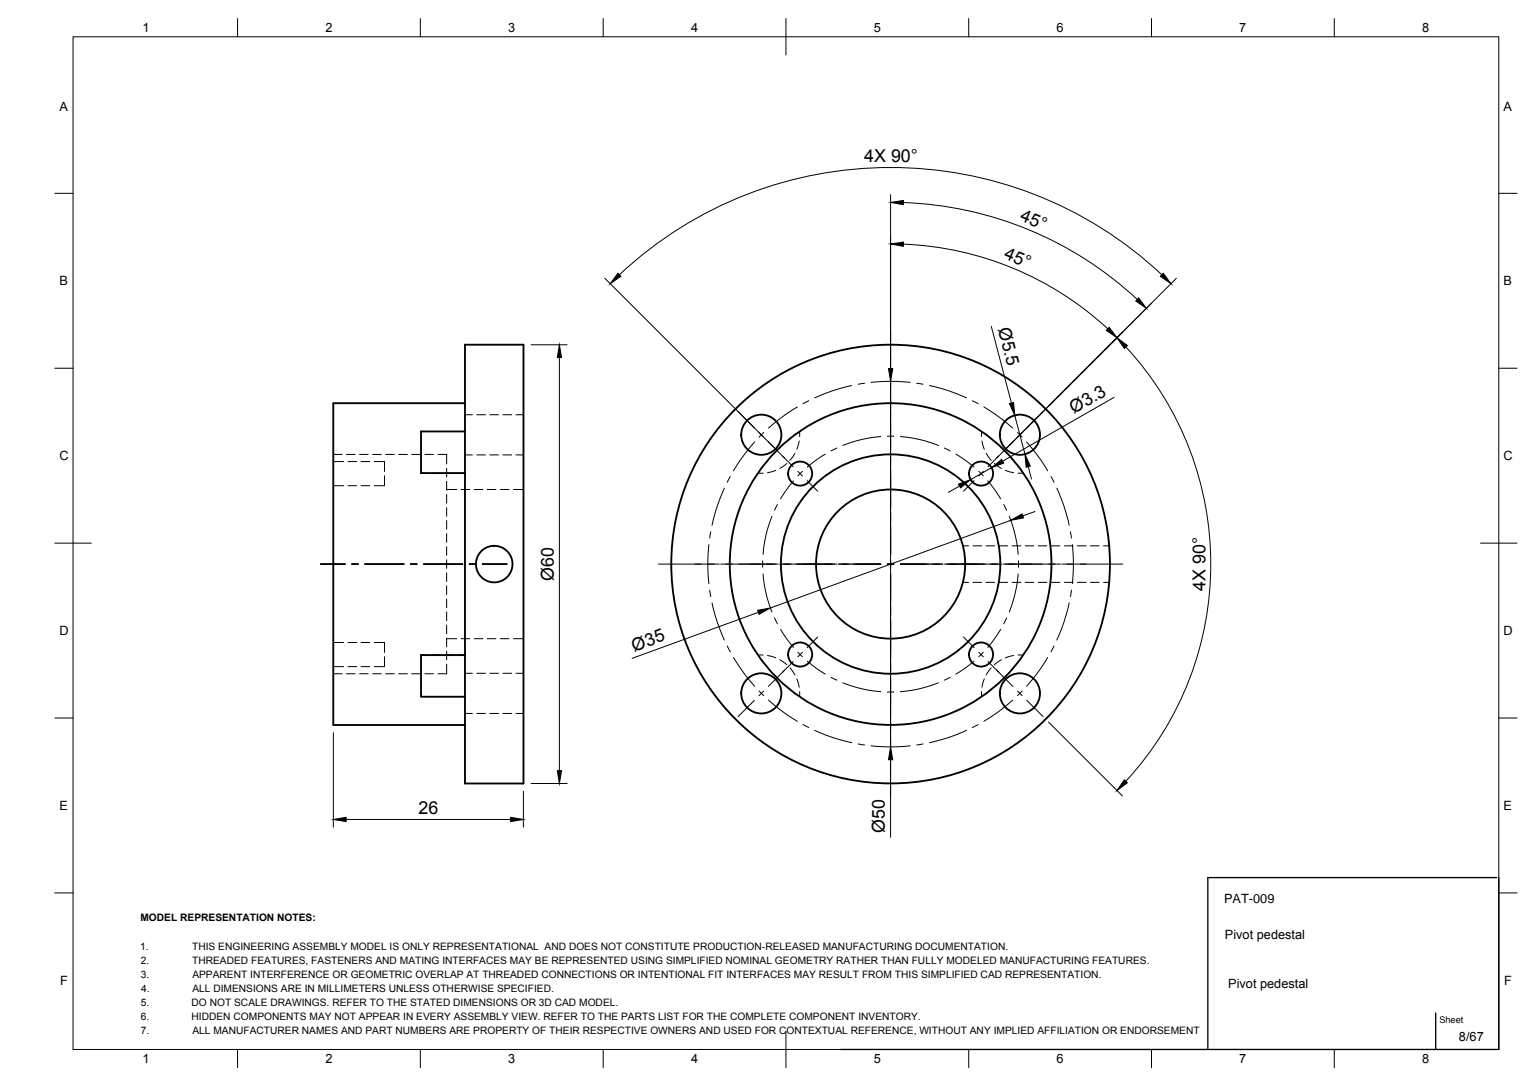
ISO-10303-21;
HEADER;
/* Generated by software containing ST-Developer
 * from STEP Tools, Inc. (www.steptools.com) 
 */

FILE_DESCRIPTION(
/* description */ ('Bell-crank linkage with push rods'),
/* implementation_level */ '2;1');

FILE_NAME(
/* name */ 'Pivot pedestal.step',
/* time_stamp */ '2026-10-28T03:25:15-07:00',
/* author */ (''),
/* organization */ (''),
/* preprocessor_version */ 'ST-DEVELOPER v20.2',
/* originating_system */ 'Autodesk Translation Framework v15.17.0.0',
/* authorisation */ '');

FILE_SCHEMA (('AUTOMOTIVE_DESIGN { 1 0 10303 214 3 1 1 }'));
ENDSEC;

DATA;
#10=MECHANICAL_DESIGN_GEOMETRIC_PRESENTATION_REPRESENTATION('',(#607),#16678);
#457=B_SPLINE_CURVE_WITH_KNOTS('',3,(#13690,#13691,#13692,#13693,#13694,
#13695,#13696,#13697,#13698,#13699),.UNSPECIFIED.,.F.,.F.,(4,2,2,2,4),(0.,
0.0945941824764479,0.189188364952896,0.283770357603024,0.378352350253152),
 .UNSPECIFIED.);
#458=B_SPLINE_CURVE_WITH_KNOTS('',3,(#13700,#13701,#13702,#13703,#13704,
#13705,#13706,#13707,#13708,#13709,#13710,#13711,#13712,#13713,#13714,#13715,
#13716,#13717,#13718,#13719,#13720,#13721,#13722,#13723,#13724,#13725),
 .UNSPECIFIED.,.F.,.F.,(4,2,2,2,2,2,2,2,2,2,2,2,4),(0.378352350253152,0.47293434290328,
0.567516335553408,0.662110518029855,0.756704700506303,0.851298882982751,
0.945893065459199,1.04047505810933,1.13505705075946,1.22963904340958,1.32422103605971,
1.41881521853616,1.51340940101261),.UNSPECIFIED.);
#459=B_SPLINE_CURVE_WITH_KNOTS('',3,(#13729,#13730,#13731,#13732,#13733,
#13734,#13735,#13736,#13737,#13738,#13739,#13740,#13741,#13742,#13743,#13744,
#13745,#13746,#13747,#13748,#13749,#13750,#13751,#13752,#13753,#13754),
 .UNSPECIFIED.,.F.,.F.,(4,2,2,2,2,2,2,2,2,2,2,2,4),(0.,0.0942186410044058,
0.188437282008812,0.282655768798837,0.376874255588861,0.471092742378886,
0.565311229168911,0.659529870173317,0.753748511177723,0.847967152182129,
0.942185793186535,1.03640427997656,1.13062276676658),.UNSPECIFIED.);
#460=B_SPLINE_CURVE_WITH_KNOTS('',3,(#13755,#13756,#13757,#13758,#13759,
#13760,#13761,#13762,#13763,#13764),.UNSPECIFIED.,.F.,.F.,(4,2,2,2,4),(1.13062276676658,
1.22484125355661,1.31905974034663,1.41327838135104,1.50749702235545),
 .UNSPECIFIED.);
#499=SHAPE_REPRESENTATION_RELATIONSHIP('SRR','None',#16915,#553);
#553=ADVANCED_BREP_SHAPE_REPRESENTATION('',(#669),#16620);
#607=STYLED_ITEM('',(#17305),#669);
#669=MANIFOLD_SOLID_BREP('Body1',#8797);
#749=FACE_BOUND('',#1842,.T.);
#750=FACE_BOUND('',#1843,.T.);
#751=FACE_BOUND('',#1844,.T.);
#752=FACE_BOUND('',#1845,.T.);
#753=FACE_BOUND('',#1846,.T.);
#754=FACE_BOUND('',#1853,.T.);
#755=FACE_BOUND('',#1855,.T.);
#756=FACE_BOUND('',#1857,.T.);
#757=FACE_BOUND('',#1859,.T.);
#758=FACE_BOUND('',#1860,.T.);
#759=FACE_BOUND('',#1861,.T.);
#760=FACE_BOUND('',#1862,.T.);
#761=FACE_BOUND('',#1863,.T.);
#762=FACE_BOUND('',#1865,.T.);
#763=FACE_BOUND('',#1866,.T.);
#764=FACE_BOUND('',#1867,.T.);
#765=FACE_BOUND('',#1868,.T.);
#766=FACE_BOUND('',#1869,.T.);
#984=PLANE('',#9518);
#985=PLANE('',#9522);
#986=PLANE('',#9526);
#987=PLANE('',#9530);
#988=PLANE('',#9531);
#989=PLANE('',#9539);
#990=PLANE('',#9544);
#991=PLANE('',#9549);
#992=PLANE('',#9558);
#993=PLANE('',#9575);
#994=PLANE('',#9581);
#995=PLANE('',#9582);
#1277=FACE_OUTER_BOUND('',#1823,.T.);
#1278=FACE_OUTER_BOUND('',#1824,.T.);
#1279=FACE_OUTER_BOUND('',#1825,.T.);
#1280=FACE_OUTER_BOUND('',#1826,.T.);
#1281=FACE_OUTER_BOUND('',#1827,.T.);
#1282=FACE_OUTER_BOUND('',#1828,.T.);
#1283=FACE_OUTER_BOUND('',#1829,.T.);
#1284=FACE_OUTER_BOUND('',#1830,.T.);
#1285=FACE_OUTER_BOUND('',#1831,.T.);
#1286=FACE_OUTER_BOUND('',#1832,.T.);
#1287=FACE_OUTER_BOUND('',#1833,.T.);
#1288=FACE_OUTER_BOUND('',#1834,.T.);
#1289=FACE_OUTER_BOUND('',#1835,.T.);
#1290=FACE_OUTER_BOUND('',#1836,.T.);
#1291=FACE_OUTER_BOUND('',#1837,.T.);
#1292=FACE_OUTER_BOUND('',#1838,.T.);
#1293=FACE_OUTER_BOUND('',#1839,.T.);
#1294=FACE_OUTER_BOUND('',#1840,.T.);
#1295=FACE_OUTER_BOUND('',#1841,.T.);
#1296=FACE_OUTER_BOUND('',#1847,.T.);
#1297=FACE_OUTER_BOUND('',#1848,.T.);
#1298=FACE_OUTER_BOUND('',#1849,.T.);
#1299=FACE_OUTER_BOUND('',#1850,.T.);
#1300=FACE_OUTER_BOUND('',#1851,.T.);
#1301=FACE_OUTER_BOUND('',#1852,.T.);
#1302=FACE_OUTER_BOUND('',#1854,.T.);
#1303=FACE_OUTER_BOUND('',#1856,.T.);
#1304=FACE_OUTER_BOUND('',#1858,.T.);
#1305=FACE_OUTER_BOUND('',#1864,.T.);
#1823=EDGE_LOOP('',(#6055,#6056,#6057,#6058,#6059,#6060));
#1824=EDGE_LOOP('',(#6061,#6062,#6063,#6064));
#1825=EDGE_LOOP('',(#6065));
#1826=EDGE_LOOP('',(#6066,#6067,#6068,#6069));
#1827=EDGE_LOOP('',(#6070));
#1828=EDGE_LOOP('',(#6071,#6072,#6073,#6074));
#1829=EDGE_LOOP('',(#6075));
#1830=EDGE_LOOP('',(#6076,#6077,#6078,#6079));
#1831=EDGE_LOOP('',(#6080));
#1832=EDGE_LOOP('',(#6081,#6082));
#1833=EDGE_LOOP('',(#6083,#6084,#6085,#6086));
#1834=EDGE_LOOP('',(#6087,#6088,#6089,#6090));
#1835=EDGE_LOOP('',(#6091,#6092));
#1836=EDGE_LOOP('',(#6093,#6094,#6095,#6096));
#1837=EDGE_LOOP('',(#6097,#6098));
#1838=EDGE_LOOP('',(#6099,#6100,#6101,#6102));
#1839=EDGE_LOOP('',(#6103,#6104));
#1840=EDGE_LOOP('',(#6105,#6106,#6107,#6108,#6109,#6110,#6111,#6112,#6113,
#6114,#6115,#6116,#6117,#6118,#6119,#6120,#6121,#6122,#6123,#6124));
#1841=EDGE_LOOP('',(#6125));
#1842=EDGE_LOOP('',(#6126,#6127,#6128,#6129,#6130,#6131,#6132,#6133,#6134));
#1843=EDGE_LOOP('',(#6135));
#1844=EDGE_LOOP('',(#6136));
#1845=EDGE_LOOP('',(#6137));
#1846=EDGE_LOOP('',(#6138));
#1847=EDGE_LOOP('',(#6139,#6140,#6141,#6142));
#1848=EDGE_LOOP('',(#6143,#6144,#6145,#6146));
#1849=EDGE_LOOP('',(#6147,#6148,#6149,#6150));
#1850=EDGE_LOOP('',(#6151,#6152,#6153,#6154));
#1851=EDGE_LOOP('',(#6155,#6156,#6157,#6158));
#1852=EDGE_LOOP('',(#6159));
#1853=EDGE_LOOP('',(#6160));
#1854=EDGE_LOOP('',(#6161,#6162,#6163,#6164));
#1855=EDGE_LOOP('',(#6165,#6166));
#1856=EDGE_LOOP('',(#6167,#6168,#6169,#6170));
#1857=EDGE_LOOP('',(#6171,#6172));
#1858=EDGE_LOOP('',(#6173));
#1859=EDGE_LOOP('',(#6174));
#1860=EDGE_LOOP('',(#6175));
#1861=EDGE_LOOP('',(#6176));
#1862=EDGE_LOOP('',(#6177));
#1863=EDGE_LOOP('',(#6178));
#1864=EDGE_LOOP('',(#6179));
#1865=EDGE_LOOP('',(#6180));
#1866=EDGE_LOOP('',(#6181));
#1867=EDGE_LOOP('',(#6182));
#1868=EDGE_LOOP('',(#6183));
#1869=EDGE_LOOP('',(#6184));
#2580=LINE('',#13727,#3129);
#2581=LINE('',#13769,#3130);
#2582=LINE('',#13776,#3131);
#2583=LINE('',#13783,#3132);
#2584=LINE('',#13790,#3133);
#2585=LINE('',#13800,#3134);
#2586=LINE('',#13803,#3135);
#2587=LINE('',#13807,#3136);
#2588=LINE('',#13811,#3137);
#2589=LINE('',#13818,#3138);
#2590=LINE('',#13822,#3139);
#2591=LINE('',#13829,#3140);
#2592=LINE('',#13833,#3141);
#2593=LINE('',#13841,#3142);
#2594=LINE('',#13861,#3143);
#2595=LINE('',#13865,#3144);
#2596=LINE('',#13869,#3145);
#2597=LINE('',#13873,#3146);
#2598=LINE('',#13878,#3147);
#2599=LINE('',#13885,#3148);
#2600=LINE('',#13889,#3149);
#3129=VECTOR('',#10800,0.25);
#3130=VECTOR('',#10805,0.165);
#3131=VECTOR('',#10814,0.165);
#3132=VECTOR('',#10823,0.165);
#3133=VECTOR('',#10832,0.165);
#3134=VECTOR('',#10845,1.);
#3135=VECTOR('',#10848,1.);
#3136=VECTOR('',#10851,1.);
#3137=VECTOR('',#10854,1.);
#3138=VECTOR('',#10863,1.);
#3139=VECTOR('',#10866,1.);
#3140=VECTOR('',#10875,1.);
#3141=VECTOR('',#10878,1.);
#3142=VECTOR('',#10889,2.2);
#3143=VECTOR('',#10916,0.275);
#3144=VECTOR('',#10921,0.275);
#3145=VECTOR('',#10926,0.275);
#3146=VECTOR('',#10931,0.275);
#3147=VECTOR('',#10936,1.5);
#3148=VECTOR('',#10945,3.);
#3149=VECTOR('',#10950,1.02);
#3654=CIRCLE('',#9516,0.165);
#3655=CIRCLE('',#9517,0.165);
#3656=CIRCLE('',#9520,0.165);
#3657=CIRCLE('',#9521,0.165);
#3658=CIRCLE('',#9524,0.165);
#3659=CIRCLE('',#9525,0.165);
#3660=CIRCLE('',#9528,0.165);
#3661=CIRCLE('',#9529,0.165);
#3662=CIRCLE('',#9532,2.2);
#3663=CIRCLE('',#9533,0.525);
#3664=CIRCLE('',#9535,0.525);
#3665=CIRCLE('',#9537,0.525);
#3666=CIRCLE('',#9538,0.525);
#3667=CIRCLE('',#9540,2.2);
#3668=CIRCLE('',#9542,0.525);
#3669=CIRCLE('',#9543,0.525);
#3670=CIRCLE('',#9545,2.2);
#3671=CIRCLE('',#9547,0.525);
#3672=CIRCLE('',#9548,0.525);
#3673=CIRCLE('',#9550,2.2);
#3674=CIRCLE('',#9552,2.2);
#3675=CIRCLE('',#9553,2.2);
#3676=CIRCLE('',#9554,2.2);
#3677=CIRCLE('',#9555,2.2);
#3678=CIRCLE('',#9556,2.2);
#3679=CIRCLE('',#9557,2.2);
#3680=CIRCLE('',#9559,3.);
#3681=CIRCLE('',#9560,0.275);
#3682=CIRCLE('',#9561,0.275);
#3683=CIRCLE('',#9562,0.275);
#3684=CIRCLE('',#9563,0.275);
#3685=CIRCLE('',#9565,0.275);
#3686=CIRCLE('',#9567,0.275);
#3687=CIRCLE('',#9569,0.275);
#3688=CIRCLE('',#9571,0.275);
#3689=CIRCLE('',#9573,1.5);
#3690=CIRCLE('',#9574,1.5);
#3691=CIRCLE('',#9576,1.02);
#3692=CIRCLE('',#9578,3.);
#3693=CIRCLE('',#9580,1.02);
#4168=VERTEX_POINT('',#13688);
#4169=VERTEX_POINT('',#13689);
#4170=VERTEX_POINT('',#13726);
#4171=VERTEX_POINT('',#13728);
#4172=VERTEX_POINT('',#13766);
#4173=VERTEX_POINT('',#13768);
#4174=VERTEX_POINT('',#13773);
#4175=VERTEX_POINT('',#13775);
#4176=VERTEX_POINT('',#13780);
#4177=VERTEX_POINT('',#13782);
#4178=VERTEX_POINT('',#13787);
#4179=VERTEX_POINT('',#13789);
#4180=VERTEX_POINT('',#13794);
#4181=VERTEX_POINT('',#13795);
#4182=VERTEX_POINT('',#13799);
#4183=VERTEX_POINT('',#13801);
#4184=VERTEX_POINT('',#13805);
#4185=VERTEX_POINT('',#13806);
#4186=VERTEX_POINT('',#13808);
#4187=VERTEX_POINT('',#13810);
#4188=VERTEX_POINT('',#13816);
#4189=VERTEX_POINT('',#13817);
#4190=VERTEX_POINT('',#13819);
#4191=VERTEX_POINT('',#13821);
#4192=VERTEX_POINT('',#13827);
#4193=VERTEX_POINT('',#13828);
#4194=VERTEX_POINT('',#13830);
#4195=VERTEX_POINT('',#13832);
#4196=VERTEX_POINT('',#13838);
#4197=VERTEX_POINT('',#13840);
#4198=VERTEX_POINT('',#13848);
#4199=VERTEX_POINT('',#13850);
#4200=VERTEX_POINT('',#13852);
#4201=VERTEX_POINT('',#13854);
#4202=VERTEX_POINT('',#13856);
#4203=VERTEX_POINT('',#13859);
#4204=VERTEX_POINT('',#13863);
#4205=VERTEX_POINT('',#13867);
#4206=VERTEX_POINT('',#13871);
#4207=VERTEX_POINT('',#13875);
#4208=VERTEX_POINT('',#13877);
#4209=VERTEX_POINT('',#13881);
#4210=VERTEX_POINT('',#13884);
#4211=VERTEX_POINT('',#13888);
#4905=EDGE_CURVE('',#4168,#4169,#457,.T.);
#4906=EDGE_CURVE('',#4169,#4168,#458,.T.);
#4907=EDGE_CURVE('',#4169,#4170,#2580,.T.);
#4908=EDGE_CURVE('',#4171,#4170,#459,.T.);
#4909=EDGE_CURVE('',#4170,#4171,#460,.T.);
#4910=EDGE_CURVE('',#4172,#4172,#3654,.T.);
#4911=EDGE_CURVE('',#4172,#4173,#2581,.T.);
#4912=EDGE_CURVE('',#4173,#4173,#3655,.T.);
#4913=EDGE_CURVE('',#4174,#4174,#3656,.T.);
#4914=EDGE_CURVE('',#4174,#4175,#2582,.T.);
#4915=EDGE_CURVE('',#4175,#4175,#3657,.T.);
#4916=EDGE_CURVE('',#4176,#4176,#3658,.T.);
#4917=EDGE_CURVE('',#4176,#4177,#2583,.T.);
#4918=EDGE_CURVE('',#4177,#4177,#3659,.T.);
#4919=EDGE_CURVE('',#4178,#4178,#3660,.T.);
#4920=EDGE_CURVE('',#4178,#4179,#2584,.T.);
#4921=EDGE_CURVE('',#4179,#4179,#3661,.T.);
#4922=EDGE_CURVE('',#4180,#4181,#3662,.T.);
#4923=EDGE_CURVE('',#4181,#4180,#3663,.T.);
#4924=EDGE_CURVE('',#4182,#4180,#2585,.T.);
#4925=EDGE_CURVE('',#4183,#4182,#3664,.T.);
#4926=EDGE_CURVE('',#4181,#4183,#2586,.T.);
#4927=EDGE_CURVE('',#4184,#4185,#2587,.T.);
#4928=EDGE_CURVE('',#4184,#4186,#3665,.T.);
#4929=EDGE_CURVE('',#4187,#4186,#2588,.T.);
#4930=EDGE_CURVE('',#4185,#4187,#3666,.T.);
#4931=EDGE_CURVE('',#4186,#4184,#3667,.T.);
#4932=EDGE_CURVE('',#4188,#4189,#2589,.T.);
#4933=EDGE_CURVE('',#4188,#4190,#3668,.T.);
#4934=EDGE_CURVE('',#4191,#4190,#2590,.T.);
#4935=EDGE_CURVE('',#4189,#4191,#3669,.T.);
#4936=EDGE_CURVE('',#4190,#4188,#3670,.T.);
#4937=EDGE_CURVE('',#4192,#4193,#2591,.T.);
#4938=EDGE_CURVE('',#4192,#4194,#3671,.T.);
#4939=EDGE_CURVE('',#4195,#4194,#2592,.T.);
#4940=EDGE_CURVE('',#4193,#4195,#3672,.T.);
#4941=EDGE_CURVE('',#4194,#4192,#3673,.T.);
#4942=EDGE_CURVE('',#4196,#4196,#3674,.T.);
#4943=EDGE_CURVE('',#4196,#4197,#2593,.T.);
#4944=EDGE_CURVE('',#4197,#4182,#3675,.T.);
#4945=EDGE_CURVE('',#4183,#4195,#3676,.T.);
#4946=EDGE_CURVE('',#4193,#4191,#3677,.T.);
#4947=EDGE_CURVE('',#4189,#4187,#3678,.T.);
#4948=EDGE_CURVE('',#4185,#4197,#3679,.T.);
#4949=EDGE_CURVE('',#4198,#4198,#3680,.T.);
#4950=EDGE_CURVE('',#4199,#4199,#3681,.T.);
#4951=EDGE_CURVE('',#4200,#4200,#3682,.T.);
#4952=EDGE_CURVE('',#4201,#4201,#3683,.T.);
#4953=EDGE_CURVE('',#4202,#4202,#3684,.T.);
#4954=EDGE_CURVE('',#4203,#4203,#3685,.T.);
#4955=EDGE_CURVE('',#4203,#4199,#2594,.T.);
#4956=EDGE_CURVE('',#4204,#4204,#3686,.T.);
#4957=EDGE_CURVE('',#4204,#4202,#2595,.T.);
#4958=EDGE_CURVE('',#4205,#4205,#3687,.T.);
#4959=EDGE_CURVE('',#4205,#4200,#2596,.T.);
#4960=EDGE_CURVE('',#4206,#4206,#3688,.T.);
#4961=EDGE_CURVE('',#4206,#4201,#2597,.T.);
#4962=EDGE_CURVE('',#4207,#4207,#3689,.T.);
#4963=EDGE_CURVE('',#4207,#4208,#2598,.T.);
#4964=EDGE_CURVE('',#4208,#4208,#3690,.T.);
#4965=EDGE_CURVE('',#4209,#4209,#3691,.T.);
#4966=EDGE_CURVE('',#4198,#4210,#2599,.T.);
#4967=EDGE_CURVE('',#4210,#4210,#3692,.T.);
#4968=EDGE_CURVE('',#4209,#4211,#2600,.T.);
#4969=EDGE_CURVE('',#4211,#4211,#3693,.T.);
#6055=ORIENTED_EDGE('',*,*,#4905,.F.);
#6056=ORIENTED_EDGE('',*,*,#4906,.F.);
#6057=ORIENTED_EDGE('',*,*,#4907,.T.);
#6058=ORIENTED_EDGE('',*,*,#4908,.F.);
#6059=ORIENTED_EDGE('',*,*,#4909,.F.);
#6060=ORIENTED_EDGE('',*,*,#4907,.F.);
#6061=ORIENTED_EDGE('',*,*,#4910,.F.);
#6062=ORIENTED_EDGE('',*,*,#4911,.T.);
#6063=ORIENTED_EDGE('',*,*,#4912,.F.);
#6064=ORIENTED_EDGE('',*,*,#4911,.F.);
#6065=ORIENTED_EDGE('',*,*,#4910,.T.);
#6066=ORIENTED_EDGE('',*,*,#4913,.F.);
#6067=ORIENTED_EDGE('',*,*,#4914,.T.);
#6068=ORIENTED_EDGE('',*,*,#4915,.F.);
#6069=ORIENTED_EDGE('',*,*,#4914,.F.);
#6070=ORIENTED_EDGE('',*,*,#4913,.T.);
#6071=ORIENTED_EDGE('',*,*,#4916,.F.);
#6072=ORIENTED_EDGE('',*,*,#4917,.T.);
#6073=ORIENTED_EDGE('',*,*,#4918,.F.);
#6074=ORIENTED_EDGE('',*,*,#4917,.F.);
#6075=ORIENTED_EDGE('',*,*,#4916,.T.);
#6076=ORIENTED_EDGE('',*,*,#4919,.F.);
#6077=ORIENTED_EDGE('',*,*,#4920,.T.);
#6078=ORIENTED_EDGE('',*,*,#4921,.F.);
#6079=ORIENTED_EDGE('',*,*,#4920,.F.);
#6080=ORIENTED_EDGE('',*,*,#4919,.T.);
#6081=ORIENTED_EDGE('',*,*,#4922,.F.);
#6082=ORIENTED_EDGE('',*,*,#4923,.F.);
#6083=ORIENTED_EDGE('',*,*,#4924,.F.);
#6084=ORIENTED_EDGE('',*,*,#4925,.F.);
#6085=ORIENTED_EDGE('',*,*,#4926,.F.);
#6086=ORIENTED_EDGE('',*,*,#4923,.T.);
#6087=ORIENTED_EDGE('',*,*,#4927,.F.);
#6088=ORIENTED_EDGE('',*,*,#4928,.T.);
#6089=ORIENTED_EDGE('',*,*,#4929,.F.);
#6090=ORIENTED_EDGE('',*,*,#4930,.F.);
#6091=ORIENTED_EDGE('',*,*,#4931,.F.);
#6092=ORIENTED_EDGE('',*,*,#4928,.F.);
#6093=ORIENTED_EDGE('',*,*,#4932,.F.);
#6094=ORIENTED_EDGE('',*,*,#4933,.T.);
#6095=ORIENTED_EDGE('',*,*,#4934,.F.);
#6096=ORIENTED_EDGE('',*,*,#4935,.F.);
#6097=ORIENTED_EDGE('',*,*,#4936,.F.);
#6098=ORIENTED_EDGE('',*,*,#4933,.F.);
#6099=ORIENTED_EDGE('',*,*,#4937,.F.);
#6100=ORIENTED_EDGE('',*,*,#4938,.T.);
#6101=ORIENTED_EDGE('',*,*,#4939,.F.);
#6102=ORIENTED_EDGE('',*,*,#4940,.F.);
#6103=ORIENTED_EDGE('',*,*,#4941,.F.);
#6104=ORIENTED_EDGE('',*,*,#4938,.F.);
#6105=ORIENTED_EDGE('',*,*,#4942,.F.);
#6106=ORIENTED_EDGE('',*,*,#4943,.T.);
#6107=ORIENTED_EDGE('',*,*,#4944,.T.);
#6108=ORIENTED_EDGE('',*,*,#4924,.T.);
#6109=ORIENTED_EDGE('',*,*,#4922,.T.);
#6110=ORIENTED_EDGE('',*,*,#4926,.T.);
#6111=ORIENTED_EDGE('',*,*,#4945,.T.);
#6112=ORIENTED_EDGE('',*,*,#4939,.T.);
#6113=ORIENTED_EDGE('',*,*,#4941,.T.);
#6114=ORIENTED_EDGE('',*,*,#4937,.T.);
#6115=ORIENTED_EDGE('',*,*,#4946,.T.);
#6116=ORIENTED_EDGE('',*,*,#4934,.T.);
#6117=ORIENTED_EDGE('',*,*,#4936,.T.);
#6118=ORIENTED_EDGE('',*,*,#4932,.T.);
#6119=ORIENTED_EDGE('',*,*,#4947,.T.);
#6120=ORIENTED_EDGE('',*,*,#4929,.T.);
#6121=ORIENTED_EDGE('',*,*,#4931,.T.);
#6122=ORIENTED_EDGE('',*,*,#4927,.T.);
#6123=ORIENTED_EDGE('',*,*,#4948,.T.);
#6124=ORIENTED_EDGE('',*,*,#4943,.F.);
#6125=ORIENTED_EDGE('',*,*,#4949,.T.);
#6126=ORIENTED_EDGE('',*,*,#4948,.F.);
#6127=ORIENTED_EDGE('',*,*,#4930,.T.);
#6128=ORIENTED_EDGE('',*,*,#4947,.F.);
#6129=ORIENTED_EDGE('',*,*,#4935,.T.);
#6130=ORIENTED_EDGE('',*,*,#4946,.F.);
#6131=ORIENTED_EDGE('',*,*,#4940,.T.);
#6132=ORIENTED_EDGE('',*,*,#4945,.F.);
#6133=ORIENTED_EDGE('',*,*,#4925,.T.);
#6134=ORIENTED_EDGE('',*,*,#4944,.F.);
#6135=ORIENTED_EDGE('',*,*,#4950,.T.);
#6136=ORIENTED_EDGE('',*,*,#4951,.T.);
#6137=ORIENTED_EDGE('',*,*,#4952,.T.);
#6138=ORIENTED_EDGE('',*,*,#4953,.T.);
#6139=ORIENTED_EDGE('',*,*,#4954,.F.);
#6140=ORIENTED_EDGE('',*,*,#4955,.T.);
#6141=ORIENTED_EDGE('',*,*,#4950,.F.);
#6142=ORIENTED_EDGE('',*,*,#4955,.F.);
#6143=ORIENTED_EDGE('',*,*,#4956,.F.);
#6144=ORIENTED_EDGE('',*,*,#4957,.T.);
#6145=ORIENTED_EDGE('',*,*,#4953,.F.);
#6146=ORIENTED_EDGE('',*,*,#4957,.F.);
#6147=ORIENTED_EDGE('',*,*,#4958,.F.);
#6148=ORIENTED_EDGE('',*,*,#4959,.T.);
#6149=ORIENTED_EDGE('',*,*,#4951,.F.);
#6150=ORIENTED_EDGE('',*,*,#4959,.F.);
#6151=ORIENTED_EDGE('',*,*,#4960,.F.);
#6152=ORIENTED_EDGE('',*,*,#4961,.T.);
#6153=ORIENTED_EDGE('',*,*,#4952,.F.);
#6154=ORIENTED_EDGE('',*,*,#4961,.F.);
#6155=ORIENTED_EDGE('',*,*,#4962,.F.);
#6156=ORIENTED_EDGE('',*,*,#4963,.T.);
#6157=ORIENTED_EDGE('',*,*,#4964,.F.);
#6158=ORIENTED_EDGE('',*,*,#4963,.F.);
#6159=ORIENTED_EDGE('',*,*,#4962,.T.);
#6160=ORIENTED_EDGE('',*,*,#4965,.F.);
#6161=ORIENTED_EDGE('',*,*,#4949,.F.);
#6162=ORIENTED_EDGE('',*,*,#4966,.T.);
#6163=ORIENTED_EDGE('',*,*,#4967,.T.);
#6164=ORIENTED_EDGE('',*,*,#4966,.F.);
#6165=ORIENTED_EDGE('',*,*,#4908,.T.);
#6166=ORIENTED_EDGE('',*,*,#4909,.T.);
#6167=ORIENTED_EDGE('',*,*,#4965,.T.);
#6168=ORIENTED_EDGE('',*,*,#4968,.T.);
#6169=ORIENTED_EDGE('',*,*,#4969,.T.);
#6170=ORIENTED_EDGE('',*,*,#4968,.F.);
#6171=ORIENTED_EDGE('',*,*,#4905,.T.);
#6172=ORIENTED_EDGE('',*,*,#4906,.T.);
#6173=ORIENTED_EDGE('',*,*,#4942,.T.);
#6174=ORIENTED_EDGE('',*,*,#4964,.T.);
#6175=ORIENTED_EDGE('',*,*,#4921,.T.);
#6176=ORIENTED_EDGE('',*,*,#4918,.T.);
#6177=ORIENTED_EDGE('',*,*,#4915,.T.);
#6178=ORIENTED_EDGE('',*,*,#4912,.T.);
#6179=ORIENTED_EDGE('',*,*,#4967,.F.);
#6180=ORIENTED_EDGE('',*,*,#4969,.F.);
#6181=ORIENTED_EDGE('',*,*,#4960,.T.);
#6182=ORIENTED_EDGE('',*,*,#4958,.T.);
#6183=ORIENTED_EDGE('',*,*,#4956,.T.);
#6184=ORIENTED_EDGE('',*,*,#4954,.T.);
#8079=CYLINDRICAL_SURFACE('',#9514,0.25);
#8080=CYLINDRICAL_SURFACE('',#9515,0.165);
#8081=CYLINDRICAL_SURFACE('',#9519,0.165);
#8082=CYLINDRICAL_SURFACE('',#9523,0.165);
#8083=CYLINDRICAL_SURFACE('',#9527,0.165);
#8084=CYLINDRICAL_SURFACE('',#9534,0.525);
#8085=CYLINDRICAL_SURFACE('',#9536,0.525);
#8086=CYLINDRICAL_SURFACE('',#9541,0.525);
#8087=CYLINDRICAL_SURFACE('',#9546,0.525);
#8088=CYLINDRICAL_SURFACE('',#9551,2.2);
#8089=CYLINDRICAL_SURFACE('',#9564,0.275);
#8090=CYLINDRICAL_SURFACE('',#9566,0.275);
#8091=CYLINDRICAL_SURFACE('',#9568,0.275);
#8092=CYLINDRICAL_SURFACE('',#9570,0.275);
#8093=CYLINDRICAL_SURFACE('',#9572,1.5);
#8094=CYLINDRICAL_SURFACE('',#9577,3.);
#8095=CYLINDRICAL_SURFACE('',#9579,1.02);
#8302=ADVANCED_FACE('',(#1277),#8079,.F.);
#8303=ADVANCED_FACE('',(#1278),#8080,.F.);
#8304=ADVANCED_FACE('',(#1279),#984,.T.);
#8305=ADVANCED_FACE('',(#1280),#8081,.F.);
#8306=ADVANCED_FACE('',(#1281),#985,.T.);
#8307=ADVANCED_FACE('',(#1282),#8082,.F.);
#8308=ADVANCED_FACE('',(#1283),#986,.T.);
#8309=ADVANCED_FACE('',(#1284),#8083,.F.);
#8310=ADVANCED_FACE('',(#1285),#987,.T.);
#8311=ADVANCED_FACE('',(#1286),#988,.F.);
#8312=ADVANCED_FACE('',(#1287),#8084,.F.);
#8313=ADVANCED_FACE('',(#1288),#8085,.F.);
#8314=ADVANCED_FACE('',(#1289),#989,.F.);
#8315=ADVANCED_FACE('',(#1290),#8086,.F.);
#8316=ADVANCED_FACE('',(#1291),#990,.F.);
#8317=ADVANCED_FACE('',(#1292),#8087,.F.);
#8318=ADVANCED_FACE('',(#1293),#991,.F.);
#8319=ADVANCED_FACE('',(#1294),#8088,.T.);
#8320=ADVANCED_FACE('',(#1295,#749,#750,#751,#752,#753),#992,.T.);
#8321=ADVANCED_FACE('',(#1296),#8089,.F.);
#8322=ADVANCED_FACE('',(#1297),#8090,.F.);
#8323=ADVANCED_FACE('',(#1298),#8091,.F.);
#8324=ADVANCED_FACE('',(#1299),#8092,.F.);
#8325=ADVANCED_FACE('',(#1300),#8093,.F.);
#8326=ADVANCED_FACE('',(#1301,#754),#993,.T.);
#8327=ADVANCED_FACE('',(#1302,#755),#8094,.T.);
#8328=ADVANCED_FACE('',(#1303,#756),#8095,.F.);
#8329=ADVANCED_FACE('',(#1304,#757,#758,#759,#760,#761),#994,.T.);
#8330=ADVANCED_FACE('',(#1305,#762,#763,#764,#765,#766),#995,.F.);
#8797=CLOSED_SHELL('',(#8302,#8303,#8304,#8305,#8306,#8307,#8308,#8309,
#8310,#8311,#8312,#8313,#8314,#8315,#8316,#8317,#8318,#8319,#8320,#8321,
#8322,#8323,#8324,#8325,#8326,#8327,#8328,#8329,#8330));
#9513=AXIS2_PLACEMENT_3D('',#13686,#10796,#10797);
#9514=AXIS2_PLACEMENT_3D('',#13687,#10798,#10799);
#9515=AXIS2_PLACEMENT_3D('',#13765,#10801,#10802);
#9516=AXIS2_PLACEMENT_3D('',#13767,#10803,#10804);
#9517=AXIS2_PLACEMENT_3D('',#13770,#10806,#10807);
#9518=AXIS2_PLACEMENT_3D('',#13771,#10808,#10809);
#9519=AXIS2_PLACEMENT_3D('',#13772,#10810,#10811);
#9520=AXIS2_PLACEMENT_3D('',#13774,#10812,#10813);
#9521=AXIS2_PLACEMENT_3D('',#13777,#10815,#10816);
#9522=AXIS2_PLACEMENT_3D('',#13778,#10817,#10818);
#9523=AXIS2_PLACEMENT_3D('',#13779,#10819,#10820);
#9524=AXIS2_PLACEMENT_3D('',#13781,#10821,#10822);
#9525=AXIS2_PLACEMENT_3D('',#13784,#10824,#10825);
#9526=AXIS2_PLACEMENT_3D('',#13785,#10826,#10827);
#9527=AXIS2_PLACEMENT_3D('',#13786,#10828,#10829);
#9528=AXIS2_PLACEMENT_3D('',#13788,#10830,#10831);
#9529=AXIS2_PLACEMENT_3D('',#13791,#10833,#10834);
#9530=AXIS2_PLACEMENT_3D('',#13792,#10835,#10836);
#9531=AXIS2_PLACEMENT_3D('',#13793,#10837,#10838);
#9532=AXIS2_PLACEMENT_3D('',#13796,#10839,#10840);
#9533=AXIS2_PLACEMENT_3D('',#13797,#10841,#10842);
#9534=AXIS2_PLACEMENT_3D('',#13798,#10843,#10844);
#9535=AXIS2_PLACEMENT_3D('',#13802,#10846,#10847);
#9536=AXIS2_PLACEMENT_3D('',#13804,#10849,#10850);
#9537=AXIS2_PLACEMENT_3D('',#13809,#10852,#10853);
#9538=AXIS2_PLACEMENT_3D('',#13812,#10855,#10856);
#9539=AXIS2_PLACEMENT_3D('',#13813,#10857,#10858);
#9540=AXIS2_PLACEMENT_3D('',#13814,#10859,#10860);
#9541=AXIS2_PLACEMENT_3D('',#13815,#10861,#10862);
#9542=AXIS2_PLACEMENT_3D('',#13820,#10864,#10865);
#9543=AXIS2_PLACEMENT_3D('',#13823,#10867,#10868);
#9544=AXIS2_PLACEMENT_3D('',#13824,#10869,#10870);
#9545=AXIS2_PLACEMENT_3D('',#13825,#10871,#10872);
#9546=AXIS2_PLACEMENT_3D('',#13826,#10873,#10874);
#9547=AXIS2_PLACEMENT_3D('',#13831,#10876,#10877);
#9548=AXIS2_PLACEMENT_3D('',#13834,#10879,#10880);
#9549=AXIS2_PLACEMENT_3D('',#13835,#10881,#10882);
#9550=AXIS2_PLACEMENT_3D('',#13836,#10883,#10884);
#9551=AXIS2_PLACEMENT_3D('',#13837,#10885,#10886);
#9552=AXIS2_PLACEMENT_3D('',#13839,#10887,#10888);
#9553=AXIS2_PLACEMENT_3D('',#13842,#10890,#10891);
#9554=AXIS2_PLACEMENT_3D('',#13843,#10892,#10893);
#9555=AXIS2_PLACEMENT_3D('',#13844,#10894,#10895);
#9556=AXIS2_PLACEMENT_3D('',#13845,#10896,#10897);
#9557=AXIS2_PLACEMENT_3D('',#13846,#10898,#10899);
#9558=AXIS2_PLACEMENT_3D('',#13847,#10900,#10901);
#9559=AXIS2_PLACEMENT_3D('',#13849,#10902,#10903);
#9560=AXIS2_PLACEMENT_3D('',#13851,#10904,#10905);
#9561=AXIS2_PLACEMENT_3D('',#13853,#10906,#10907);
#9562=AXIS2_PLACEMENT_3D('',#13855,#10908,#10909);
#9563=AXIS2_PLACEMENT_3D('',#13857,#10910,#10911);
#9564=AXIS2_PLACEMENT_3D('',#13858,#10912,#10913);
#9565=AXIS2_PLACEMENT_3D('',#13860,#10914,#10915);
#9566=AXIS2_PLACEMENT_3D('',#13862,#10917,#10918);
#9567=AXIS2_PLACEMENT_3D('',#13864,#10919,#10920);
#9568=AXIS2_PLACEMENT_3D('',#13866,#10922,#10923);
#9569=AXIS2_PLACEMENT_3D('',#13868,#10924,#10925);
#9570=AXIS2_PLACEMENT_3D('',#13870,#10927,#10928);
#9571=AXIS2_PLACEMENT_3D('',#13872,#10929,#10930);
#9572=AXIS2_PLACEMENT_3D('',#13874,#10932,#10933);
#9573=AXIS2_PLACEMENT_3D('',#13876,#10934,#10935);
#9574=AXIS2_PLACEMENT_3D('',#13879,#10937,#10938);
#9575=AXIS2_PLACEMENT_3D('',#13880,#10939,#10940);
#9576=AXIS2_PLACEMENT_3D('',#13882,#10941,#10942);
#9577=AXIS2_PLACEMENT_3D('',#13883,#10943,#10944);
#9578=AXIS2_PLACEMENT_3D('',#13886,#10946,#10947);
#9579=AXIS2_PLACEMENT_3D('',#13887,#10948,#10949);
#9580=AXIS2_PLACEMENT_3D('',#13890,#10951,#10952);
#9581=AXIS2_PLACEMENT_3D('',#13891,#10953,#10954);
#9582=AXIS2_PLACEMENT_3D('',#13892,#10955,#10956);
#10796=DIRECTION('axis',(0.,0.,1.));
#10797=DIRECTION('refdir',(1.,0.,0.));
#10798=DIRECTION('center_axis',(1.,0.,0.));
#10799=DIRECTION('ref_axis',(0.,0.,-1.));
#10800=DIRECTION('',(1.,0.,0.));
#10801=DIRECTION('center_axis',(0.,0.,1.));
#10802=DIRECTION('ref_axis',(1.,0.,0.));
#10803=DIRECTION('center_axis',(0.,0.,1.));
#10804=DIRECTION('ref_axis',(1.,0.,0.));
#10805=DIRECTION('',(0.,0.,1.));
#10806=DIRECTION('center_axis',(0.,0.,-1.));
#10807=DIRECTION('ref_axis',(1.,0.,0.));
#10808=DIRECTION('center_axis',(0.,0.,1.));
#10809=DIRECTION('ref_axis',(1.,0.,0.));
#10810=DIRECTION('center_axis',(0.,0.,1.));
#10811=DIRECTION('ref_axis',(1.,0.,0.));
#10812=DIRECTION('center_axis',(0.,0.,1.));
#10813=DIRECTION('ref_axis',(1.,0.,0.));
#10814=DIRECTION('',(0.,0.,1.));
#10815=DIRECTION('center_axis',(0.,0.,-1.));
#10816=DIRECTION('ref_axis',(1.,0.,0.));
#10817=DIRECTION('center_axis',(0.,0.,1.));
#10818=DIRECTION('ref_axis',(1.,0.,0.));
#10819=DIRECTION('center_axis',(0.,0.,1.));
#10820=DIRECTION('ref_axis',(1.,0.,0.));
#10821=DIRECTION('center_axis',(0.,0.,1.));
#10822=DIRECTION('ref_axis',(1.,0.,0.));
#10823=DIRECTION('',(0.,0.,1.));
#10824=DIRECTION('center_axis',(0.,0.,-1.));
#10825=DIRECTION('ref_axis',(1.,0.,0.));
#10826=DIRECTION('center_axis',(0.,0.,1.));
#10827=DIRECTION('ref_axis',(1.,0.,0.));
#10828=DIRECTION('center_axis',(0.,0.,1.));
#10829=DIRECTION('ref_axis',(1.,0.,0.));
#10830=DIRECTION('center_axis',(0.,0.,1.));
#10831=DIRECTION('ref_axis',(1.,0.,0.));
#10832=DIRECTION('',(0.,0.,1.));
#10833=DIRECTION('center_axis',(0.,0.,-1.));
#10834=DIRECTION('ref_axis',(1.,0.,0.));
#10835=DIRECTION('center_axis',(0.,0.,1.));
#10836=DIRECTION('ref_axis',(1.,0.,0.));
#10837=DIRECTION('center_axis',(0.,0.,1.));
#10838=DIRECTION('ref_axis',(1.,0.,0.));
#10839=DIRECTION('center_axis',(0.,0.,1.));
#10840=DIRECTION('ref_axis',(1.,0.,0.));
#10841=DIRECTION('center_axis',(0.,0.,1.));
#10842=DIRECTION('ref_axis',(1.,0.,0.));
#10843=DIRECTION('center_axis',(0.,0.,1.));
#10844=DIRECTION('ref_axis',(1.,0.,0.));
#10845=DIRECTION('',(0.,0.,1.));
#10846=DIRECTION('center_axis',(0.,0.,1.));
#10847=DIRECTION('ref_axis',(1.,0.,0.));
#10848=DIRECTION('',(0.,0.,-1.));
#10849=DIRECTION('center_axis',(0.,0.,1.));
#10850=DIRECTION('ref_axis',(1.,0.,0.));
#10851=DIRECTION('',(0.,0.,-1.));
#10852=DIRECTION('center_axis',(0.,0.,1.));
#10853=DIRECTION('ref_axis',(1.,0.,0.));
#10854=DIRECTION('',(0.,0.,1.));
#10855=DIRECTION('center_axis',(0.,0.,1.));
#10856=DIRECTION('ref_axis',(1.,0.,0.));
#10857=DIRECTION('center_axis',(0.,0.,1.));
#10858=DIRECTION('ref_axis',(1.,0.,0.));
#10859=DIRECTION('center_axis',(0.,0.,1.));
#10860=DIRECTION('ref_axis',(1.,0.,0.));
#10861=DIRECTION('center_axis',(0.,0.,1.));
#10862=DIRECTION('ref_axis',(-0.707106781186548,-0.707106781186547,0.));
#10863=DIRECTION('',(0.,0.,-1.));
#10864=DIRECTION('center_axis',(0.,0.,1.));
#10865=DIRECTION('ref_axis',(1.,0.,0.));
#10866=DIRECTION('',(0.,0.,1.));
#10867=DIRECTION('center_axis',(0.,0.,1.));
#10868=DIRECTION('ref_axis',(1.,0.,0.));
#10869=DIRECTION('center_axis',(0.,0.,1.));
#10870=DIRECTION('ref_axis',(1.,0.,0.));
#10871=DIRECTION('center_axis',(0.,0.,1.));
#10872=DIRECTION('ref_axis',(1.,0.,0.));
#10873=DIRECTION('center_axis',(0.,0.,1.));
#10874=DIRECTION('ref_axis',(-0.707106781186547,0.707106781186548,0.));
#10875=DIRECTION('',(0.,0.,-1.));
#10876=DIRECTION('center_axis',(0.,0.,1.));
#10877=DIRECTION('ref_axis',(1.,0.,0.));
#10878=DIRECTION('',(0.,0.,1.));
#10879=DIRECTION('center_axis',(0.,0.,1.));
#10880=DIRECTION('ref_axis',(1.,0.,0.));
#10881=DIRECTION('center_axis',(0.,0.,1.));
#10882=DIRECTION('ref_axis',(1.,0.,0.));
#10883=DIRECTION('center_axis',(0.,0.,1.));
#10884=DIRECTION('ref_axis',(1.,0.,0.));
#10885=DIRECTION('center_axis',(0.,0.,1.));
#10886=DIRECTION('ref_axis',(1.,0.,0.));
#10887=DIRECTION('center_axis',(0.,0.,1.));
#10888=DIRECTION('ref_axis',(1.,0.,0.));
#10889=DIRECTION('',(0.,0.,-1.));
#10890=DIRECTION('center_axis',(0.,0.,1.));
#10891=DIRECTION('ref_axis',(1.,0.,0.));
#10892=DIRECTION('center_axis',(0.,0.,1.));
#10893=DIRECTION('ref_axis',(1.,0.,0.));
#10894=DIRECTION('center_axis',(0.,0.,1.));
#10895=DIRECTION('ref_axis',(1.,0.,0.));
#10896=DIRECTION('center_axis',(0.,0.,1.));
#10897=DIRECTION('ref_axis',(1.,0.,0.));
#10898=DIRECTION('center_axis',(0.,0.,1.));
#10899=DIRECTION('ref_axis',(1.,0.,0.));
#10900=DIRECTION('center_axis',(0.,0.,1.));
#10901=DIRECTION('ref_axis',(1.,0.,0.));
#10902=DIRECTION('center_axis',(0.,0.,1.));
#10903=DIRECTION('ref_axis',(1.,0.,0.));
#10904=DIRECTION('center_axis',(0.,0.,-1.));
#10905=DIRECTION('ref_axis',(1.,0.,0.));
#10906=DIRECTION('center_axis',(0.,0.,-1.));
#10907=DIRECTION('ref_axis',(1.,0.,0.));
#10908=DIRECTION('center_axis',(0.,0.,-1.));
#10909=DIRECTION('ref_axis',(1.,0.,0.));
#10910=DIRECTION('center_axis',(0.,0.,-1.));
#10911=DIRECTION('ref_axis',(1.,0.,0.));
#10912=DIRECTION('center_axis',(0.,0.,1.));
#10913=DIRECTION('ref_axis',(1.,0.,0.));
#10914=DIRECTION('center_axis',(0.,0.,1.));
#10915=DIRECTION('ref_axis',(1.,0.,0.));
#10916=DIRECTION('',(0.,0.,1.));
#10917=DIRECTION('center_axis',(0.,0.,1.));
#10918=DIRECTION('ref_axis',(1.,0.,0.));
#10919=DIRECTION('center_axis',(0.,0.,1.));
#10920=DIRECTION('ref_axis',(1.,0.,0.));
#10921=DIRECTION('',(0.,0.,1.));
#10922=DIRECTION('center_axis',(0.,0.,1.));
#10923=DIRECTION('ref_axis',(1.,0.,0.));
#10924=DIRECTION('center_axis',(0.,0.,1.));
#10925=DIRECTION('ref_axis',(1.,0.,0.));
#10926=DIRECTION('',(0.,0.,1.));
#10927=DIRECTION('center_axis',(0.,0.,1.));
#10928=DIRECTION('ref_axis',(1.,0.,0.));
#10929=DIRECTION('center_axis',(0.,0.,1.));
#10930=DIRECTION('ref_axis',(1.,0.,0.));
#10931=DIRECTION('',(0.,0.,1.));
#10932=DIRECTION('center_axis',(0.,0.,1.));
#10933=DIRECTION('ref_axis',(1.,0.,0.));
#10934=DIRECTION('center_axis',(0.,0.,1.));
#10935=DIRECTION('ref_axis',(1.,0.,0.));
#10936=DIRECTION('',(0.,0.,1.));
#10937=DIRECTION('center_axis',(0.,0.,-1.));
#10938=DIRECTION('ref_axis',(1.,0.,0.));
#10939=DIRECTION('center_axis',(0.,0.,1.));
#10940=DIRECTION('ref_axis',(1.,0.,0.));
#10941=DIRECTION('center_axis',(0.,0.,1.));
#10942=DIRECTION('ref_axis',(1.,0.,0.));
#10943=DIRECTION('center_axis',(0.,0.,1.));
#10944=DIRECTION('ref_axis',(1.,0.,0.));
#10945=DIRECTION('',(0.,0.,-1.));
#10946=DIRECTION('center_axis',(0.,0.,1.));
#10947=DIRECTION('ref_axis',(1.,0.,0.));
#10948=DIRECTION('center_axis',(0.,0.,1.));
#10949=DIRECTION('ref_axis',(1.,0.,0.));
#10950=DIRECTION('',(0.,0.,-1.));
#10951=DIRECTION('center_axis',(0.,0.,-1.));
#10952=DIRECTION('ref_axis',(1.,0.,0.));
#10953=DIRECTION('center_axis',(0.,0.,1.));
#10954=DIRECTION('ref_axis',(1.,0.,0.));
#10955=DIRECTION('center_axis',(0.,0.,1.));
#10956=DIRECTION('ref_axis',(1.,0.,0.));
#13686=CARTESIAN_POINT('',(0.,0.,0.));
#13687=CARTESIAN_POINT('Origin',(0.9,0.,1.4));
#13688=CARTESIAN_POINT('',(0.988888264668966,0.25,1.4));
#13689=CARTESIAN_POINT('',(1.02,-1.18386380373883E-17,1.65));
#13690=CARTESIAN_POINT('Ctrl Pts',(0.988888264668966,0.25,1.4));
#13691=CARTESIAN_POINT('Ctrl Pts',(0.988888264668966,0.25,1.43153139415882));
#13692=CARTESIAN_POINT('Ctrl Pts',(0.990553370646674,0.243672048431404,
1.46507214966317));
#13693=CARTESIAN_POINT('Ctrl Pts',(0.996491737296663,0.218119830014375,
1.52662620974954));
#13694=CARTESIAN_POINT('Ctrl Pts',(1.00067109353237,0.198902128206072,1.5546512623872));
#13695=CARTESIAN_POINT('Ctrl Pts',(1.00845756932386,0.154654113568716,1.59889927702456));
#13696=CARTESIAN_POINT('Ctrl Pts',(1.01258144235289,0.126627870945253,1.61811920309393));
#13697=CARTESIAN_POINT('Ctrl Pts',(1.0183917429657,0.065069600391363,1.64367304400768));
#13698=CARTESIAN_POINT('Ctrl Pts',(1.02,0.031527330883376,1.65));
#13699=CARTESIAN_POINT('Ctrl Pts',(1.02,2.77555756156289E-17,1.65));
#13700=CARTESIAN_POINT('Ctrl Pts',(1.02,6.93889390390723E-18,1.65));
#13701=CARTESIAN_POINT('Ctrl Pts',(1.02,-0.031527330883376,1.65));
#13702=CARTESIAN_POINT('Ctrl Pts',(1.0183917429657,-0.065069600391363,1.64367304400768));
#13703=CARTESIAN_POINT('Ctrl Pts',(1.01258144235289,-0.126627870945253,
1.61811920309393));
#13704=CARTESIAN_POINT('Ctrl Pts',(1.00845756932386,-0.154654113568716,
1.59889927702456));
#13705=CARTESIAN_POINT('Ctrl Pts',(1.00067109353237,-0.198902128206072,
1.5546512623872));
#13706=CARTESIAN_POINT('Ctrl Pts',(0.996491737296663,-0.218119830014375,
1.52662620974954));
#13707=CARTESIAN_POINT('Ctrl Pts',(0.990553370646674,-0.243672048431404,
1.46507214966317));
#13708=CARTESIAN_POINT('Ctrl Pts',(0.988888264668967,-0.25,1.43153139415882));
#13709=CARTESIAN_POINT('Ctrl Pts',(0.988888264668967,-0.25,1.36846860584118));
#13710=CARTESIAN_POINT('Ctrl Pts',(0.990553370646674,-0.243672048431404,
1.33492785033683));
#13711=CARTESIAN_POINT('Ctrl Pts',(0.996491737296663,-0.218119830014375,
1.27337379025046));
#13712=CARTESIAN_POINT('Ctrl Pts',(1.00067109353237,-0.198902128206072,
1.2453487376128));
#13713=CARTESIAN_POINT('Ctrl Pts',(1.00845756932386,-0.154654113568716,
1.20110072297544));
#13714=CARTESIAN_POINT('Ctrl Pts',(1.01258144235289,-0.126627870945254,
1.18188079690607));
#13715=CARTESIAN_POINT('Ctrl Pts',(1.0183917429657,-0.0650696003913633,
1.15632695599232));
#13716=CARTESIAN_POINT('Ctrl Pts',(1.02,-0.0315273308833761,1.15));
#13717=CARTESIAN_POINT('Ctrl Pts',(1.02,0.0315273308833759,1.15));
#13718=CARTESIAN_POINT('Ctrl Pts',(1.0183917429657,0.065069600391363,1.15632695599232));
#13719=CARTESIAN_POINT('Ctrl Pts',(1.01258144235289,0.126627870945253,1.18188079690607));
#13720=CARTESIAN_POINT('Ctrl Pts',(1.00845756932386,0.154654113568716,1.20110072297544));
#13721=CARTESIAN_POINT('Ctrl Pts',(1.00067109353237,0.198902128206072,1.2453487376128));
#13722=CARTESIAN_POINT('Ctrl Pts',(0.996491737296663,0.218119830014375,
1.27337379025046));
#13723=CARTESIAN_POINT('Ctrl Pts',(0.990553370646674,0.243672048431404,
1.33492785033683));
#13724=CARTESIAN_POINT('Ctrl Pts',(0.988888264668967,0.25,1.36846860584118));
#13725=CARTESIAN_POINT('Ctrl Pts',(0.988888264668967,0.25,1.4));
#13726=CARTESIAN_POINT('',(3.,-3.06161699786838E-17,1.65));
#13727=CARTESIAN_POINT('',(0.9,-3.06161699786838E-17,1.65));
#13728=CARTESIAN_POINT('',(2.98956518577535,0.25,1.4));
#13729=CARTESIAN_POINT('Ctrl Pts',(2.98956518577535,0.25,1.4));
#13730=CARTESIAN_POINT('Ctrl Pts',(2.98956518577535,0.25,1.36859378633186));
#13731=CARTESIAN_POINT('Ctrl Pts',(2.99011104995181,0.24372047740942,1.33510417960069));
#13732=CARTESIAN_POINT('Ctrl Pts',(2.99208145165098,0.218202539734559,1.27351367328886));
#13733=CARTESIAN_POINT('Ctrl Pts',(2.99347740802958,0.198964922639276,1.245411532046));
#13734=CARTESIAN_POINT('Ctrl Pts',(2.99609686518216,0.154588504271054,1.20103511367778));
#13735=CARTESIAN_POINT('Ctrl Pts',(2.99749070376198,0.126486346986081,1.18179746841036));
#13736=CARTESIAN_POINT('Ctrl Pts',(2.99945625936844,0.0648957875009219,
1.15627950921557));
#13737=CARTESIAN_POINT('Ctrl Pts',(3.,0.0314061622633416,1.15));
#13738=CARTESIAN_POINT('Ctrl Pts',(3.,-0.0314061622633416,1.15));
#13739=CARTESIAN_POINT('Ctrl Pts',(2.99945625936844,-0.0648957875009221,
1.15627950921557));
#13740=CARTESIAN_POINT('Ctrl Pts',(2.99749070376198,-0.126486346986081,
1.18179746841036));
#13741=CARTESIAN_POINT('Ctrl Pts',(2.99609686518216,-0.154588504271054,
1.20103511367778));
#13742=CARTESIAN_POINT('Ctrl Pts',(2.99347740802958,-0.198964922639276,
1.245411532046));
#13743=CARTESIAN_POINT('Ctrl Pts',(2.99208145165098,-0.218202539734559,
1.27351367328886));
#13744=CARTESIAN_POINT('Ctrl Pts',(2.99011104995181,-0.24372047740942,1.33510417960069));
#13745=CARTESIAN_POINT('Ctrl Pts',(2.98956518577535,-0.25,1.36859378633186));
#13746=CARTESIAN_POINT('Ctrl Pts',(2.98956518577535,-0.25,1.43140621366814));
#13747=CARTESIAN_POINT('Ctrl Pts',(2.99011104995181,-0.24372047740942,1.4648958203993));
#13748=CARTESIAN_POINT('Ctrl Pts',(2.99208145165098,-0.21820253973456,1.52648632671114));
#13749=CARTESIAN_POINT('Ctrl Pts',(2.99347740802958,-0.198964922639276,
1.554588467954));
#13750=CARTESIAN_POINT('Ctrl Pts',(2.99609686518216,-0.154588504271054,
1.59896488632222));
#13751=CARTESIAN_POINT('Ctrl Pts',(2.99749070376198,-0.126486346986082,
1.61820253158964));
#13752=CARTESIAN_POINT('Ctrl Pts',(2.99945625936844,-0.0648957875009221,
1.64372049078443));
#13753=CARTESIAN_POINT('Ctrl Pts',(3.,-0.0314061622633417,1.65));
#13754=CARTESIAN_POINT('Ctrl Pts',(3.,-5.55111512312578E-17,1.65));
#13755=CARTESIAN_POINT('Ctrl Pts',(3.,-2.08166817117217E-17,1.65));
#13756=CARTESIAN_POINT('Ctrl Pts',(3.,0.0314061622633416,1.65));
#13757=CARTESIAN_POINT('Ctrl Pts',(2.99945625936844,0.0648957875009221,
1.64372049078443));
#13758=CARTESIAN_POINT('Ctrl Pts',(2.99749070376198,0.126486346986081,1.61820253158964));
#13759=CARTESIAN_POINT('Ctrl Pts',(2.99609686518216,0.154588504271054,1.59896488632222));
#13760=CARTESIAN_POINT('Ctrl Pts',(2.99347740802958,0.198964922639276,1.554588467954));
#13761=CARTESIAN_POINT('Ctrl Pts',(2.99208145165098,0.218202539734559,1.52648632671114));
#13762=CARTESIAN_POINT('Ctrl Pts',(2.99011104995181,0.24372047740942,1.46489582039931));
#13763=CARTESIAN_POINT('Ctrl Pts',(2.98956518577535,0.25,1.43140621366814));
#13764=CARTESIAN_POINT('Ctrl Pts',(2.98956518577535,0.25,1.4));
#13765=CARTESIAN_POINT('Origin',(-1.23743686707646,-1.23743686707646,2.9));
#13766=CARTESIAN_POINT('',(-1.40243686707646,-1.23743686707646,2.9));
#13767=CARTESIAN_POINT('Origin',(-1.23743686707646,-1.23743686707646,2.9));
#13768=CARTESIAN_POINT('',(-1.40243686707646,-1.23743686707646,3.6));
#13769=CARTESIAN_POINT('',(-1.40243686707646,-1.23743686707646,2.9));
#13770=CARTESIAN_POINT('Origin',(-1.23743686707646,-1.23743686707646,3.6));
#13771=CARTESIAN_POINT('Origin',(-1.23743686707646,-1.23743686707646,2.9));
#13772=CARTESIAN_POINT('Origin',(-1.23743686707646,1.23743686707646,2.9));
#13773=CARTESIAN_POINT('',(-1.40243686707646,1.23743686707646,2.9));
#13774=CARTESIAN_POINT('Origin',(-1.23743686707646,1.23743686707646,2.9));
#13775=CARTESIAN_POINT('',(-1.40243686707646,1.23743686707646,3.6));
#13776=CARTESIAN_POINT('',(-1.40243686707646,1.23743686707646,2.9));
#13777=CARTESIAN_POINT('Origin',(-1.23743686707646,1.23743686707646,3.6));
#13778=CARTESIAN_POINT('Origin',(-1.23743686707646,1.23743686707646,2.9));
#13779=CARTESIAN_POINT('Origin',(1.23743686707646,1.23743686707646,2.9));
#13780=CARTESIAN_POINT('',(1.07243686707646,1.23743686707646,2.9));
#13781=CARTESIAN_POINT('Origin',(1.23743686707646,1.23743686707646,2.9));
#13782=CARTESIAN_POINT('',(1.07243686707646,1.23743686707646,3.6));
#13783=CARTESIAN_POINT('',(1.07243686707646,1.23743686707646,2.9));
#13784=CARTESIAN_POINT('Origin',(1.23743686707646,1.23743686707646,3.6));
#13785=CARTESIAN_POINT('Origin',(1.23743686707646,1.23743686707646,2.9));
#13786=CARTESIAN_POINT('Origin',(1.23743686707646,-1.23743686707646,2.9));
#13787=CARTESIAN_POINT('',(1.07243686707646,-1.23743686707646,2.9));
#13788=CARTESIAN_POINT('Origin',(1.23743686707646,-1.23743686707646,2.9));
#13789=CARTESIAN_POINT('',(1.07243686707646,-1.23743686707646,3.6));
#13790=CARTESIAN_POINT('',(1.07243686707646,-1.23743686707646,2.9));
#13791=CARTESIAN_POINT('Origin',(1.23743686707646,-1.23743686707646,3.6));
#13792=CARTESIAN_POINT('Origin',(1.23743686707646,-1.23743686707646,2.9));
#13793=CARTESIAN_POINT('Origin',(-1.76776695296637,-1.76776695296637,2.4));
#13794=CARTESIAN_POINT('',(-1.8139637388702,-1.24480341984751,2.4));
#13795=CARTESIAN_POINT('',(-1.24480341984751,-1.81396373887019,2.4));
#13796=CARTESIAN_POINT('Origin',(0.,0.,2.4));
#13797=CARTESIAN_POINT('Origin',(-1.76776695296637,-1.76776695296637,2.4));
#13798=CARTESIAN_POINT('Origin',(-1.76776695296637,-1.76776695296637,1.8));
#13799=CARTESIAN_POINT('',(-1.8139637388702,-1.24480341984751,1.8));
#13800=CARTESIAN_POINT('',(-1.8139637388702,-1.24480341984751,1.8));
#13801=CARTESIAN_POINT('',(-1.24480341984751,-1.81396373887019,1.8));
#13802=CARTESIAN_POINT('Origin',(-1.76776695296637,-1.76776695296637,1.8));
#13803=CARTESIAN_POINT('',(-1.24480341984751,-1.81396373887019,1.8));
#13804=CARTESIAN_POINT('Origin',(-1.76776695296637,1.76776695296637,1.8));
#13805=CARTESIAN_POINT('',(-1.81396373887019,1.24480341984751,2.4));
#13806=CARTESIAN_POINT('',(-1.81396373887019,1.24480341984751,1.8));
#13807=CARTESIAN_POINT('',(-1.81396373887019,1.24480341984751,1.8));
#13808=CARTESIAN_POINT('',(-1.24480341984751,1.81396373887019,2.4));
#13809=CARTESIAN_POINT('Origin',(-1.76776695296637,1.76776695296637,2.4));
#13810=CARTESIAN_POINT('',(-1.24480341984751,1.81396373887019,1.8));
#13811=CARTESIAN_POINT('',(-1.24480341984751,1.81396373887019,1.8));
#13812=CARTESIAN_POINT('Origin',(-1.76776695296637,1.76776695296637,1.8));
#13813=CARTESIAN_POINT('Origin',(-1.76776695296637,1.76776695296637,2.4));
#13814=CARTESIAN_POINT('Origin',(0.,0.,2.4));
#13815=CARTESIAN_POINT('Origin',(1.76776695296637,1.76776695296637,1.8));
#13816=CARTESIAN_POINT('',(1.24480341984751,1.81396373887019,2.4));
#13817=CARTESIAN_POINT('',(1.24480341984751,1.81396373887019,1.8));
#13818=CARTESIAN_POINT('',(1.24480341984751,1.81396373887019,1.8));
#13819=CARTESIAN_POINT('',(1.81396373887019,1.24480341984751,2.4));
#13820=CARTESIAN_POINT('Origin',(1.76776695296637,1.76776695296637,2.4));
#13821=CARTESIAN_POINT('',(1.81396373887019,1.24480341984751,1.8));
#13822=CARTESIAN_POINT('',(1.81396373887019,1.24480341984751,1.8));
#13823=CARTESIAN_POINT('Origin',(1.76776695296637,1.76776695296637,1.8));
#13824=CARTESIAN_POINT('Origin',(1.76776695296637,1.76776695296637,2.4));
#13825=CARTESIAN_POINT('Origin',(0.,0.,2.4));
#13826=CARTESIAN_POINT('Origin',(1.76776695296637,-1.76776695296637,1.8));
#13827=CARTESIAN_POINT('',(1.81396373887019,-1.24480341984751,2.4));
#13828=CARTESIAN_POINT('',(1.81396373887019,-1.24480341984751,1.8));
#13829=CARTESIAN_POINT('',(1.81396373887019,-1.24480341984751,1.8));
#13830=CARTESIAN_POINT('',(1.24480341984751,-1.8139637388702,2.4));
#13831=CARTESIAN_POINT('Origin',(1.76776695296637,-1.76776695296637,2.4));
#13832=CARTESIAN_POINT('',(1.24480341984751,-1.8139637388702,1.8));
#13833=CARTESIAN_POINT('',(1.24480341984751,-1.8139637388702,1.8));
#13834=CARTESIAN_POINT('Origin',(1.76776695296637,-1.76776695296637,1.8));
#13835=CARTESIAN_POINT('Origin',(1.76776695296637,-1.76776695296637,2.4));
#13836=CARTESIAN_POINT('Origin',(0.,0.,2.4));
#13837=CARTESIAN_POINT('Origin',(0.,0.,1.));
#13838=CARTESIAN_POINT('',(-2.2,-2.69422295812418E-16,3.6));
#13839=CARTESIAN_POINT('Origin',(0.,0.,3.6));
#13840=CARTESIAN_POINT('',(-2.2,-2.69422295812418E-16,1.8));
#13841=CARTESIAN_POINT('',(-2.2,-2.69422295812418E-16,1.));
#13842=CARTESIAN_POINT('Origin',(0.,0.,1.8));
#13843=CARTESIAN_POINT('Origin',(0.,0.,1.8));
#13844=CARTESIAN_POINT('Origin',(0.,0.,1.8));
#13845=CARTESIAN_POINT('Origin',(0.,0.,1.8));
#13846=CARTESIAN_POINT('Origin',(0.,0.,1.8));
#13847=CARTESIAN_POINT('Origin',(0.,0.,1.8));
#13848=CARTESIAN_POINT('',(-3.,-3.67394039744206E-16,1.8));
#13849=CARTESIAN_POINT('Origin',(0.,0.,1.8));
#13850=CARTESIAN_POINT('',(-2.04276695296637,-1.76776695296637,1.8));
#13851=CARTESIAN_POINT('Origin',(-1.76776695296637,-1.76776695296637,1.8));
#13852=CARTESIAN_POINT('',(1.49276695296637,1.76776695296637,1.8));
#13853=CARTESIAN_POINT('Origin',(1.76776695296637,1.76776695296637,1.8));
#13854=CARTESIAN_POINT('',(1.49276695296637,-1.76776695296637,1.8));
#13855=CARTESIAN_POINT('Origin',(1.76776695296637,-1.76776695296637,1.8));
#13856=CARTESIAN_POINT('',(-2.04276695296637,1.76776695296637,1.8));
#13857=CARTESIAN_POINT('Origin',(-1.76776695296637,1.76776695296637,1.8));
#13858=CARTESIAN_POINT('Origin',(-1.76776695296637,-1.76776695296637,0.9));
#13859=CARTESIAN_POINT('',(-2.04276695296637,-1.76776695296637,1.));
#13860=CARTESIAN_POINT('Origin',(-1.76776695296637,-1.76776695296637,1.));
#13861=CARTESIAN_POINT('',(-2.04276695296637,-1.76776695296637,0.9));
#13862=CARTESIAN_POINT('Origin',(-1.76776695296637,1.76776695296637,0.9));
#13863=CARTESIAN_POINT('',(-2.04276695296637,1.76776695296637,1.));
#13864=CARTESIAN_POINT('Origin',(-1.76776695296637,1.76776695296637,1.));
#13865=CARTESIAN_POINT('',(-2.04276695296637,1.76776695296637,0.9));
#13866=CARTESIAN_POINT('Origin',(1.76776695296637,1.76776695296637,0.9));
#13867=CARTESIAN_POINT('',(1.49276695296637,1.76776695296637,1.));
#13868=CARTESIAN_POINT('Origin',(1.76776695296637,1.76776695296637,1.));
#13869=CARTESIAN_POINT('',(1.49276695296637,1.76776695296637,0.9));
#13870=CARTESIAN_POINT('Origin',(1.76776695296637,-1.76776695296637,0.9));
#13871=CARTESIAN_POINT('',(1.49276695296637,-1.76776695296637,1.));
#13872=CARTESIAN_POINT('Origin',(1.76776695296637,-1.76776695296637,1.));
#13873=CARTESIAN_POINT('',(1.49276695296637,-1.76776695296637,0.9));
#13874=CARTESIAN_POINT('Origin',(0.,0.,2.05));
#13875=CARTESIAN_POINT('',(-1.5,-1.83697019872103E-16,2.05));
#13876=CARTESIAN_POINT('Origin',(0.,0.,2.05));
#13877=CARTESIAN_POINT('',(-1.5,1.83697019872103E-16,3.6));
#13878=CARTESIAN_POINT('',(-1.5,-1.83697019872103E-16,2.05));
#13879=CARTESIAN_POINT('Origin',(0.,0.,3.6));
#13880=CARTESIAN_POINT('Origin',(0.,0.,2.05));
#13881=CARTESIAN_POINT('',(-1.02,-1.2491397351303E-16,2.05));
#13882=CARTESIAN_POINT('Origin',(0.,0.,2.05));
#13883=CARTESIAN_POINT('Origin',(0.,0.,1.));
#13884=CARTESIAN_POINT('',(-3.,-3.67394039744206E-16,1.));
#13885=CARTESIAN_POINT('',(-3.,-3.67394039744206E-16,1.));
#13886=CARTESIAN_POINT('Origin',(0.,0.,1.));
#13887=CARTESIAN_POINT('Origin',(0.,0.,1.));
#13888=CARTESIAN_POINT('',(-1.02,-1.2491397351303E-16,1.));
#13889=CARTESIAN_POINT('',(-1.02,-1.2491397351303E-16,1.));
#13890=CARTESIAN_POINT('Origin',(0.,0.,1.));
#13891=CARTESIAN_POINT('Origin',(0.,0.,3.6));
#13892=CARTESIAN_POINT('Origin',(0.,0.,1.));
#16556=UNCERTAINTY_MEASURE_WITH_UNIT(LENGTH_MEASURE(0.001),#16679,
'DISTANCE_ACCURACY_VALUE',
'Maximum model space distance between geometric entities at asserted c
onnectivities');
#16614=UNCERTAINTY_MEASURE_WITH_UNIT(LENGTH_MEASURE(0.001),#16679,
'DISTANCE_ACCURACY_VALUE',
'Maximum model space distance between geometric entities at asserted c
onnectivities');
#16620=(
GEOMETRIC_REPRESENTATION_CONTEXT(3)
GLOBAL_UNCERTAINTY_ASSIGNED_CONTEXT((#16556))
GLOBAL_UNIT_ASSIGNED_CONTEXT((#16679,#16681,#16682))
REPRESENTATION_CONTEXT('','3D')
);
#16678=(
GEOMETRIC_REPRESENTATION_CONTEXT(3)
GLOBAL_UNCERTAINTY_ASSIGNED_CONTEXT((#16614))
GLOBAL_UNIT_ASSIGNED_CONTEXT((#16679,#16681,#16682))
REPRESENTATION_CONTEXT('','3D')
);
#16679=(
LENGTH_UNIT()
NAMED_UNIT(*)
SI_UNIT(.CENTI.,.METRE.)
);
#16681=(
NAMED_UNIT(*)
PLANE_ANGLE_UNIT()
SI_UNIT($,.RADIAN.)
);
#16682=(
NAMED_UNIT(*)
SI_UNIT($,.STERADIAN.)
SOLID_ANGLE_UNIT()
);
#16688=SHAPE_DEFINITION_REPRESENTATION(#16751,#16915);
#16751=PRODUCT_DEFINITION_SHAPE('',$,#16979);
#16915=SHAPE_REPRESENTATION('',(#9513),#16620);
#16973=PRODUCT_DEFINITION_CONTEXT('part definition',#17164,'design');
#16979=PRODUCT_DEFINITION('Pivot pedestal','Pivot pedestal',#17042,#16973);
#17042=PRODUCT_DEFINITION_FORMATION('',$,#17171);
#17164=APPLICATION_CONTEXT(
'Core Data for Automotive Mechanical Design Process');
#17165=PRODUCT_CONTEXT('part definition',#17164,'mechanical');
#17171=PRODUCT('Pivot pedestal','Pivot pedestal','Pivot pedestal',(#17165));
#17299=COLOUR_RGB('Off White',0.89,0.88,0.83);
#17300=FILL_AREA_STYLE_COLOUR('',#17299);
#17301=FILL_AREA_STYLE('',(#17300));
#17302=SURFACE_STYLE_FILL_AREA(#17301);
#17303=SURFACE_SIDE_STYLE('',(#17302));
#17304=SURFACE_STYLE_USAGE(.BOTH.,#17303);
#17305=PRESENTATION_STYLE_ASSIGNMENT((#17304));
ENDSEC;
END-ISO-10303-21;
